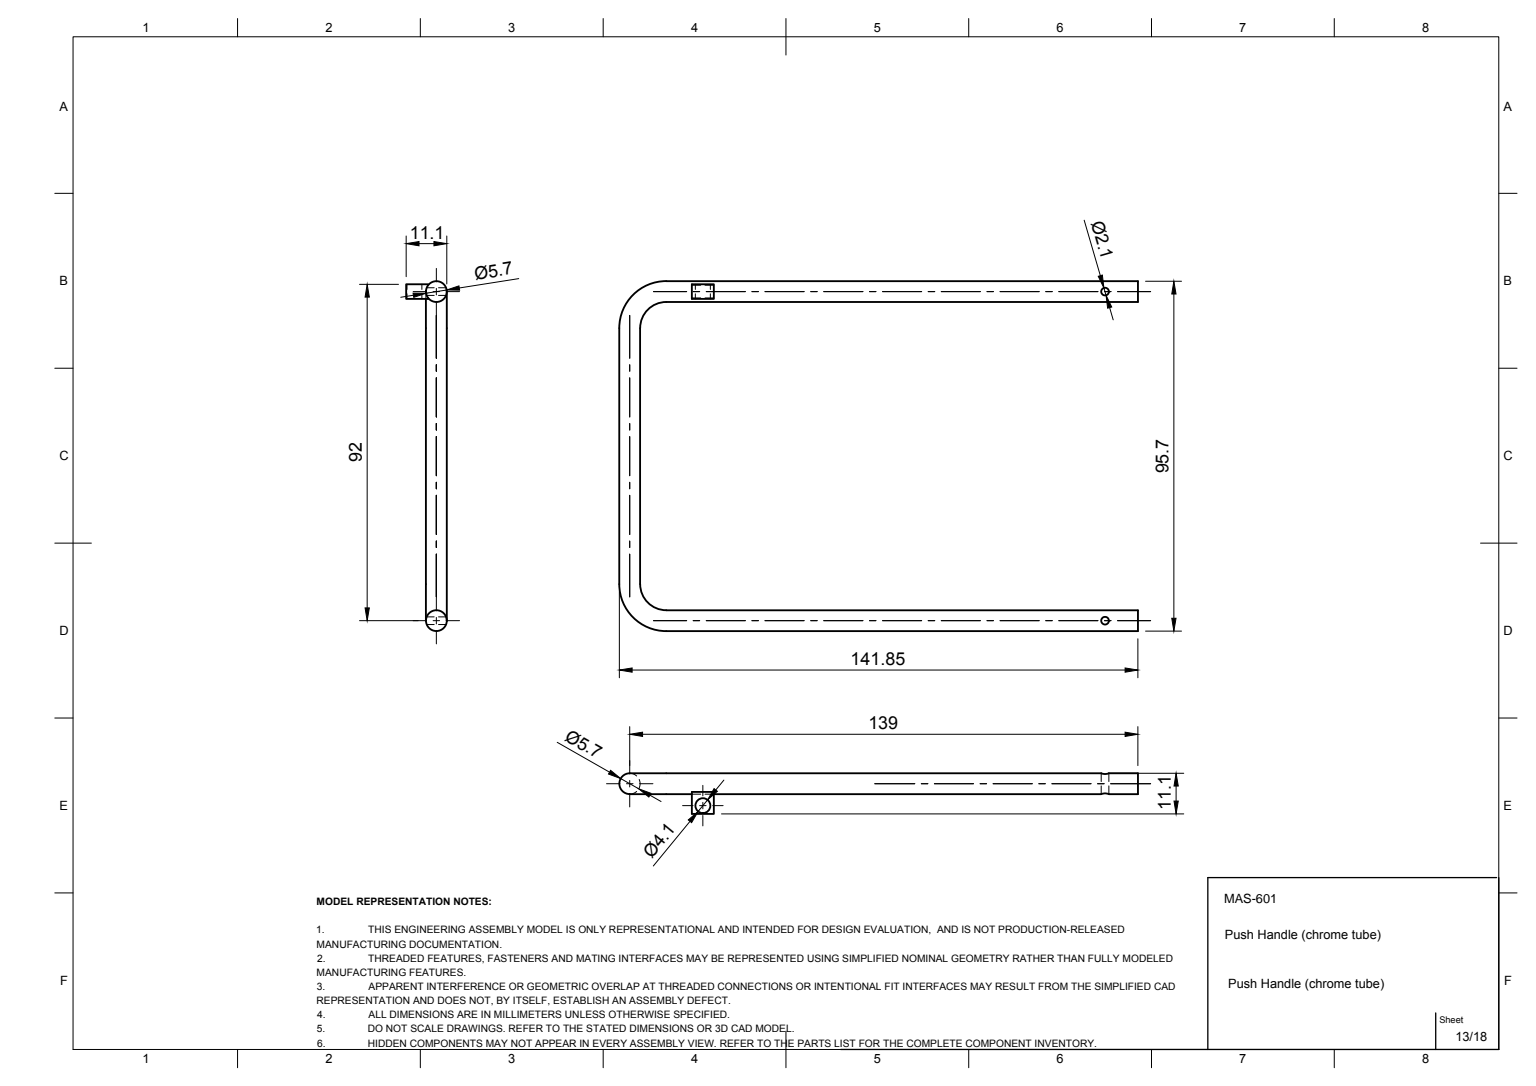
ISO-10303-21;
HEADER;
FILE_DESCRIPTION((''),'2;1');
FILE_NAME('Push Handle (chrome tube).step','2026-10-06T07:37:42+05:00',(''),(''),'','','');
FILE_SCHEMA (('AUTOMOTIVE_DESIGN { 1 0 10303 214 3 1 1 }'));
ENDSEC;
DATA;
#10=MECHANICAL_DESIGN_GEOMETRIC_PRESENTATION_REPRESENTATION('',(#381),#18757);
#335=TOROIDAL_SURFACE('',#10190,10.,2.85) ;
#336=TOROIDAL_SURFACE('',#10197,10.,2.85) ;
#347=SHAPE_REPRESENTATION_RELATIONSHIP('SRR','None',#18865,#364) ;
#364=ADVANCED_BREP_SHAPE_REPRESENTATION('',(#398),#18748) ;
#381=STYLED_ITEM('',(#18959),#398) ;
#398=MANIFOLD_SOLID_BREP('Push Handle (chrome tube)',#9550) ;
#428=B_SPLINE_CURVE_WITH_KNOTS('',3,(#14926,#14927,#14928,#14929,#14930,
#14931,#14932,#14933,#14934,#14935,#14936,#14937,#14938,#14939,#14940,#14941,
#14942,#14943),.UNSPECIFIED.,.F.,.F.,(4,2,2,2,2,2,2,2,4),(0.159853073606258,
0.199802153604227,0.239751233602197,0.279728690407356,0.319706147212516,
0.359683604017676,0.399661060822836,0.439610140820805,0.479559220818774),
 .UNSPECIFIED.) ;
#429=B_SPLINE_CURVE_WITH_KNOTS('',3,(#14944,#14945,#14946,#14947,#14948,
#14949,#14950,#14951,#14952,#14953,#14954,#14955,#14956,#14957,#14958,#14959,
#14960,#14961,#14962),.UNSPECIFIED.,.F.,.F.,(4,2,2,2,3,2,2,2,4),(0.479559220818774,
0.519508300816743,0.559457380814712,0.599434837619873,0.639412294425033,
0.679389751230192,0.719367208035352,0.759316288033321,0.799265368031291),
 .UNSPECIFIED.) ;
#430=B_SPLINE_CURVE_WITH_KNOTS('',3,(#14966,#14967,#14968,#14969,#14970,
#14971,#14972,#14973,#14974,#14975,#14976,#14977,#14978,#14979,#14980,#14981,
#14982,#14983,#14984),.UNSPECIFIED.,.F.,.F.,(4,2,2,2,3,2,2,2,4),(0.479559220818775,
0.519508300816745,0.559457380814714,0.599434837619874,0.639412294425033,
0.679389751230193,0.719367208035354,0.759316288033323,0.799265368031292),
 .UNSPECIFIED.) ;
#431=B_SPLINE_CURVE_WITH_KNOTS('',3,(#14985,#14986,#14987,#14988,#14989,
#14990,#14991,#14992,#14993,#14994,#14995,#14996,#14997,#14998,#14999,#15000,
#15001,#15002),.UNSPECIFIED.,.F.,.F.,(4,2,2,2,2,2,2,2,4),(0.159853073606259,
0.199802153604228,0.239751233602197,0.279728690407357,0.319706147212517,
0.359683604017677,0.399661060822836,0.439610140820806,0.479559220818775),
 .UNSPECIFIED.) ;
#432=B_SPLINE_CURVE_WITH_KNOTS('',3,(#15006,#15007,#15008,#15009,#15010,
#15011,#15012,#15013,#15014,#15015,#15016,#15017,#15018,#15019,#15020,#15021,
#15022,#15023),.UNSPECIFIED.,.F.,.F.,(4,2,2,2,2,2,2,2,4),(0.159853073606258,
0.199802153604227,0.239751233602197,0.279728690407356,0.319706147212516,
0.359683604017676,0.399661060822836,0.439610140820805,0.479559220818774),
 .UNSPECIFIED.) ;
#433=B_SPLINE_CURVE_WITH_KNOTS('',3,(#15027,#15028,#15029,#15030,#15031,
#15032,#15033,#15034,#15035,#15036,#15037,#15038,#15039,#15040,#15041,#15042,
#15043,#15044),.UNSPECIFIED.,.F.,.F.,(4,2,2,2,2,2,2,2,4),(0.159853073606258,
0.199802153604227,0.239751233602197,0.279728690407356,0.319706147212516,
0.359683604017676,0.399661060822836,0.439610140820805,0.479559220818774),
 .UNSPECIFIED.) ;
#434=B_SPLINE_CURVE_WITH_KNOTS('',3,(#15045,#15046,#15047,#15048,#15049,
#15050,#15051,#15052,#15053,#15054,#15055,#15056,#15057,#15058,#15059,#15060,
#15061,#15062,#15063),.UNSPECIFIED.,.F.,.F.,(4,2,2,2,3,2,2,2,4),(0.479559220818774,
0.519508300816744,0.559457380814713,0.599434837619873,0.639412294425033,
0.679389751230192,0.719367208035352,0.759316288033321,0.799265368031291),
 .UNSPECIFIED.) ;
#435=B_SPLINE_CURVE_WITH_KNOTS('',3,(#15064,#15065,#15066,#15067,#15068,
#15069,#15070,#15071,#15072,#15073,#15074,#15075,#15076,#15077,#15078,#15079,
#15080,#15081,#15082),.UNSPECIFIED.,.F.,.F.,(4,2,2,2,3,2,2,2,4),(0.479559220818774,
0.519508300816744,0.559457380814713,0.599434837619873,0.639412294425033,
0.679389751230192,0.719367208035352,0.759316288033321,0.799265368031291),
 .UNSPECIFIED.) ;
#579=CYLINDRICAL_SURFACE('',#10172,1.05) ;
#580=CYLINDRICAL_SURFACE('',#10173,1.05) ;
#581=CYLINDRICAL_SURFACE('',#10174,2.05) ;
#582=CYLINDRICAL_SURFACE('',#10186,2.85) ;
#583=CYLINDRICAL_SURFACE('',#10194,2.85) ;
#584=CYLINDRICAL_SURFACE('',#10201,2.85) ;
#722=FACE_BOUND('',#1917,.T.) ;
#723=FACE_BOUND('',#1920,.T.) ;
#724=FACE_BOUND('',#1924,.T.) ;
#725=FACE_BOUND('',#1929,.T.) ;
#726=FACE_BOUND('',#1930,.T.) ;
#893=PLANE('',#10177) ;
#894=PLANE('',#10179) ;
#895=PLANE('',#10180) ;
#896=PLANE('',#10181) ;
#897=PLANE('',#10182) ;
#898=PLANE('',#10183) ;
#899=PLANE('',#10184) ;
#900=PLANE('',#10203) ;
#901=PLANE('',#10204) ;
#1321=FACE_OUTER_BOUND('',#1911,.T.) ;
#1322=FACE_OUTER_BOUND('',#1912,.T.) ;
#1323=FACE_OUTER_BOUND('',#1913,.T.) ;
#1324=FACE_OUTER_BOUND('',#1914,.T.) ;
#1325=FACE_OUTER_BOUND('',#1915,.T.) ;
#1326=FACE_OUTER_BOUND('',#1916,.T.) ;
#1327=FACE_OUTER_BOUND('',#1918,.T.) ;
#1328=FACE_OUTER_BOUND('',#1919,.T.) ;
#1329=FACE_OUTER_BOUND('',#1921,.T.) ;
#1330=FACE_OUTER_BOUND('',#1922,.T.) ;
#1331=FACE_OUTER_BOUND('',#1923,.T.) ;
#1332=FACE_OUTER_BOUND('',#1925,.T.) ;
#1333=FACE_OUTER_BOUND('',#1926,.T.) ;
#1334=FACE_OUTER_BOUND('',#1927,.T.) ;
#1335=FACE_OUTER_BOUND('',#1928,.T.) ;
#1336=FACE_OUTER_BOUND('',#1931,.T.) ;
#1337=FACE_OUTER_BOUND('',#1932,.T.) ;
#1911=EDGE_LOOP('',(#7511,#7512,#7513,#7514,#7515,#7516)) ;
#1912=EDGE_LOOP('',(#7517,#7518,#7519,#7520,#7521,#7522)) ;
#1913=EDGE_LOOP('',(#7523,#7524,#7525,#7526)) ;
#1914=EDGE_LOOP('',(#7527,#7528,#7529,#7530,#7531,#7532)) ;
#1915=EDGE_LOOP('',(#7533,#7534,#7535,#7536)) ;
#1916=EDGE_LOOP('',(#7537,#7538,#7539,#7540)) ;
#1917=EDGE_LOOP('',(#7541)) ;
#1918=EDGE_LOOP('',(#7542,#7543,#7544,#7545)) ;
#1919=EDGE_LOOP('',(#7546,#7547,#7548,#7549)) ;
#1920=EDGE_LOOP('',(#7550)) ;
#1921=EDGE_LOOP('',(#7551,#7552,#7553,#7554)) ;
#1922=EDGE_LOOP('',(#7555,#7556,#7557,#7558,#7559,#7560)) ;
#1923=EDGE_LOOP('',(#7561,#7562,#7563,#7564,#7565,#7566,#7567,#7568,#7569)) ;
#1924=EDGE_LOOP('',(#7570,#7571)) ;
#1925=EDGE_LOOP('',(#7572,#7573,#7574,#7575,#7576,#7577)) ;
#1926=EDGE_LOOP('',(#7578,#7579,#7580,#7581,#7582,#7583)) ;
#1927=EDGE_LOOP('',(#7584,#7585,#7586,#7587,#7588,#7589)) ;
#1928=EDGE_LOOP('',(#7590,#7591,#7592,#7593,#7594,#7595,#7596,#7597,#7598)) ;
#1929=EDGE_LOOP('',(#7599,#7600)) ;
#1930=EDGE_LOOP('',(#7601,#7602,#7603,#7604)) ;
#1931=EDGE_LOOP('',(#7605)) ;
#1932=EDGE_LOOP('',(#7606)) ;
#2613=LINE('',#14964,#3384) ;
#2614=LINE('',#15025,#3385) ;
#2615=LINE('',#15087,#3386) ;
#2616=LINE('',#15094,#3387) ;
#2617=LINE('',#15096,#3388) ;
#2618=LINE('',#15098,#3389) ;
#2619=LINE('',#15100,#3390) ;
#2620=LINE('',#15101,#3391) ;
#2621=LINE('',#15104,#3392) ;
#2622=LINE('',#15106,#3393) ;
#2623=LINE('',#15107,#3394) ;
#2624=LINE('',#15111,#3395) ;
#2625=LINE('',#15112,#3396) ;
#2626=LINE('',#15113,#3397) ;
#2627=LINE('',#15116,#3398) ;
#2628=LINE('',#15117,#3399) ;
#2629=LINE('',#15119,#3400) ;
#2630=LINE('',#15122,#3401) ;
#2631=LINE('',#15123,#3402) ;
#2632=LINE('',#15129,#3403) ;
#2633=LINE('',#15131,#3404) ;
#2634=LINE('',#15143,#3405) ;
#2635=LINE('',#15154,#3406) ;
#2636=LINE('',#15156,#3407) ;
#3384=VECTOR('',#11947,1.05) ;
#3385=VECTOR('',#11950,1.05) ;
#3386=VECTOR('',#11955,2.05) ;
#3387=VECTOR('',#11962,10.) ;
#3388=VECTOR('',#11963,10.) ;
#3389=VECTOR('',#11964,10.) ;
#3390=VECTOR('',#11965,10.) ;
#3391=VECTOR('',#11966,10.) ;
#3392=VECTOR('',#11969,10.) ;
#3393=VECTOR('',#11970,10.) ;
#3394=VECTOR('',#11971,10.) ;
#3395=VECTOR('',#11974,10.) ;
#3396=VECTOR('',#11975,10.) ;
#3397=VECTOR('',#11976,10.) ;
#3398=VECTOR('',#11979,10.) ;
#3399=VECTOR('',#11980,10.) ;
#3400=VECTOR('',#11983,10.) ;
#3401=VECTOR('',#11986,10.) ;
#3402=VECTOR('',#11987,10.) ;
#3403=VECTOR('',#11996,2.85) ;
#3404=VECTOR('',#11997,2.85) ;
#3405=VECTOR('',#12012,2.85) ;
#3406=VECTOR('',#12027,2.85) ;
#3407=VECTOR('',#12028,2.85) ;
#3956=CIRCLE('',#10175,2.05) ;
#3957=CIRCLE('',#10176,2.05) ;
#3958=CIRCLE('',#10178,2.85) ;
#3959=CIRCLE('',#10185,2.85) ;
#3960=CIRCLE('',#10187,2.85) ;
#3961=CIRCLE('',#10188,2.85) ;
#3962=CIRCLE('',#10189,2.85) ;
#3963=CIRCLE('',#10191,7.15) ;
#3964=CIRCLE('',#10192,2.85) ;
#3965=CIRCLE('',#10193,2.85) ;
#3966=CIRCLE('',#10195,2.85) ;
#3967=CIRCLE('',#10196,2.85) ;
#3968=CIRCLE('',#10198,7.15000000000003) ;
#3969=CIRCLE('',#10199,2.85) ;
#3970=CIRCLE('',#10200,2.85) ;
#3971=CIRCLE('',#10202,2.85) ;
#4533=VERTEX_POINT('',#14924) ;
#4534=VERTEX_POINT('',#14925) ;
#4535=VERTEX_POINT('',#14963) ;
#4536=VERTEX_POINT('',#14965) ;
#4537=VERTEX_POINT('',#15004) ;
#4538=VERTEX_POINT('',#15005) ;
#4539=VERTEX_POINT('',#15024) ;
#4540=VERTEX_POINT('',#15026) ;
#4541=VERTEX_POINT('',#15084) ;
#4542=VERTEX_POINT('',#15086) ;
#4543=VERTEX_POINT('',#15090) ;
#4544=VERTEX_POINT('',#15091) ;
#4545=VERTEX_POINT('',#15093) ;
#4546=VERTEX_POINT('',#15095) ;
#4547=VERTEX_POINT('',#15097) ;
#4548=VERTEX_POINT('',#15099) ;
#4549=VERTEX_POINT('',#15103) ;
#4550=VERTEX_POINT('',#15105) ;
#4551=VERTEX_POINT('',#15109) ;
#4552=VERTEX_POINT('',#15110) ;
#4553=VERTEX_POINT('',#15115) ;
#4554=VERTEX_POINT('',#15121) ;
#4555=VERTEX_POINT('',#15127) ;
#4556=VERTEX_POINT('',#15130) ;
#4557=VERTEX_POINT('',#15132) ;
#4558=VERTEX_POINT('',#15136) ;
#4559=VERTEX_POINT('',#15138) ;
#4560=VERTEX_POINT('',#15142) ;
#4561=VERTEX_POINT('',#15144) ;
#4562=VERTEX_POINT('',#15148) ;
#4563=VERTEX_POINT('',#15150) ;
#4564=VERTEX_POINT('',#15155) ;
#5602=EDGE_CURVE('',#4533,#4534,#428,.T.) ;
#5603=EDGE_CURVE('',#4534,#4533,#429,.T.) ;
#5604=EDGE_CURVE('',#4534,#4535,#2613,.T.) ;
#5605=EDGE_CURVE('',#4536,#4535,#430,.T.) ;
#5606=EDGE_CURVE('',#4535,#4536,#431,.T.) ;
#5607=EDGE_CURVE('',#4537,#4538,#432,.T.) ;
#5608=EDGE_CURVE('',#4537,#4539,#2614,.T.) ;
#5609=EDGE_CURVE('',#4540,#4539,#433,.T.) ;
#5610=EDGE_CURVE('',#4539,#4540,#434,.T.) ;
#5611=EDGE_CURVE('',#4538,#4537,#435,.T.) ;
#5612=EDGE_CURVE('',#4541,#4541,#3956,.T.) ;
#5613=EDGE_CURVE('',#4541,#4542,#2615,.T.) ;
#5614=EDGE_CURVE('',#4542,#4542,#3957,.T.) ;
#5615=EDGE_CURVE('',#4543,#4544,#3958,.T.) ;
#5616=EDGE_CURVE('',#4543,#4545,#2616,.T.) ;
#5617=EDGE_CURVE('',#4545,#4546,#2617,.T.) ;
#5618=EDGE_CURVE('',#4546,#4547,#2618,.T.) ;
#5619=EDGE_CURVE('',#4547,#4548,#2619,.T.) ;
#5620=EDGE_CURVE('',#4548,#4544,#2620,.T.) ;
#5621=EDGE_CURVE('',#4549,#4543,#2621,.T.) ;
#5622=EDGE_CURVE('',#4549,#4550,#2622,.T.) ;
#5623=EDGE_CURVE('',#4550,#4545,#2623,.T.) ;
#5624=EDGE_CURVE('',#4551,#4552,#2624,.T.) ;
#5625=EDGE_CURVE('',#4552,#4548,#2625,.T.) ;
#5626=EDGE_CURVE('',#4551,#4547,#2626,.T.) ;
#5627=EDGE_CURVE('',#4553,#4551,#2627,.T.) ;
#5628=EDGE_CURVE('',#4553,#4546,#2628,.T.) ;
#5629=EDGE_CURVE('',#4550,#4553,#2629,.T.) ;
#5630=EDGE_CURVE('',#4544,#4554,#2630,.T.) ;
#5631=EDGE_CURVE('',#4552,#4554,#2631,.T.) ;
#5632=EDGE_CURVE('',#4554,#4549,#3959,.T.) ;
#5633=EDGE_CURVE('',#4555,#4555,#3960,.T.) ;
#5634=EDGE_CURVE('',#4555,#4536,#2632,.T.) ;
#5635=EDGE_CURVE('',#4535,#4556,#2633,.T.) ;
#5636=EDGE_CURVE('',#4556,#4557,#3961,.T.) ;
#5637=EDGE_CURVE('',#4557,#4556,#3962,.T.) ;
#5638=EDGE_CURVE('',#4557,#4558,#3963,.T.) ;
#5639=EDGE_CURVE('',#4558,#4559,#3964,.T.) ;
#5640=EDGE_CURVE('',#4559,#4558,#3965,.T.) ;
#5641=EDGE_CURVE('',#4559,#4560,#2634,.T.) ;
#5642=EDGE_CURVE('',#4560,#4561,#3966,.T.) ;
#5643=EDGE_CURVE('',#4561,#4560,#3967,.T.) ;
#5644=EDGE_CURVE('',#4561,#4562,#3968,.T.) ;
#5645=EDGE_CURVE('',#4562,#4563,#3969,.T.) ;
#5646=EDGE_CURVE('',#4563,#4562,#3970,.T.) ;
#5647=EDGE_CURVE('',#4563,#4539,#2635,.T.) ;
#5648=EDGE_CURVE('',#4540,#4564,#2636,.T.) ;
#5649=EDGE_CURVE('',#4564,#4564,#3971,.T.) ;
#7511=ORIENTED_EDGE('',*,*,#5602,.F.) ;
#7512=ORIENTED_EDGE('',*,*,#5603,.F.) ;
#7513=ORIENTED_EDGE('',*,*,#5604,.T.) ;
#7514=ORIENTED_EDGE('',*,*,#5605,.F.) ;
#7515=ORIENTED_EDGE('',*,*,#5606,.F.) ;
#7516=ORIENTED_EDGE('',*,*,#5604,.F.) ;
#7517=ORIENTED_EDGE('',*,*,#5607,.F.) ;
#7518=ORIENTED_EDGE('',*,*,#5608,.T.) ;
#7519=ORIENTED_EDGE('',*,*,#5609,.F.) ;
#7520=ORIENTED_EDGE('',*,*,#5610,.F.) ;
#7521=ORIENTED_EDGE('',*,*,#5608,.F.) ;
#7522=ORIENTED_EDGE('',*,*,#5611,.F.) ;
#7523=ORIENTED_EDGE('',*,*,#5612,.F.) ;
#7524=ORIENTED_EDGE('',*,*,#5613,.T.) ;
#7525=ORIENTED_EDGE('',*,*,#5614,.F.) ;
#7526=ORIENTED_EDGE('',*,*,#5613,.F.) ;
#7527=ORIENTED_EDGE('',*,*,#5615,.F.) ;
#7528=ORIENTED_EDGE('',*,*,#5616,.T.) ;
#7529=ORIENTED_EDGE('',*,*,#5617,.T.) ;
#7530=ORIENTED_EDGE('',*,*,#5618,.T.) ;
#7531=ORIENTED_EDGE('',*,*,#5619,.T.) ;
#7532=ORIENTED_EDGE('',*,*,#5620,.T.) ;
#7533=ORIENTED_EDGE('',*,*,#5621,.F.) ;
#7534=ORIENTED_EDGE('',*,*,#5622,.T.) ;
#7535=ORIENTED_EDGE('',*,*,#5623,.T.) ;
#7536=ORIENTED_EDGE('',*,*,#5616,.F.) ;
#7537=ORIENTED_EDGE('',*,*,#5624,.T.) ;
#7538=ORIENTED_EDGE('',*,*,#5625,.T.) ;
#7539=ORIENTED_EDGE('',*,*,#5619,.F.) ;
#7540=ORIENTED_EDGE('',*,*,#5626,.F.) ;
#7541=ORIENTED_EDGE('',*,*,#5614,.T.) ;
#7542=ORIENTED_EDGE('',*,*,#5627,.T.) ;
#7543=ORIENTED_EDGE('',*,*,#5626,.T.) ;
#7544=ORIENTED_EDGE('',*,*,#5618,.F.) ;
#7545=ORIENTED_EDGE('',*,*,#5628,.F.) ;
#7546=ORIENTED_EDGE('',*,*,#5629,.T.) ;
#7547=ORIENTED_EDGE('',*,*,#5628,.T.) ;
#7548=ORIENTED_EDGE('',*,*,#5617,.F.) ;
#7549=ORIENTED_EDGE('',*,*,#5623,.F.) ;
#7550=ORIENTED_EDGE('',*,*,#5612,.T.) ;
#7551=ORIENTED_EDGE('',*,*,#5630,.F.) ;
#7552=ORIENTED_EDGE('',*,*,#5620,.F.) ;
#7553=ORIENTED_EDGE('',*,*,#5625,.F.) ;
#7554=ORIENTED_EDGE('',*,*,#5631,.T.) ;
#7555=ORIENTED_EDGE('',*,*,#5632,.F.) ;
#7556=ORIENTED_EDGE('',*,*,#5631,.F.) ;
#7557=ORIENTED_EDGE('',*,*,#5624,.F.) ;
#7558=ORIENTED_EDGE('',*,*,#5627,.F.) ;
#7559=ORIENTED_EDGE('',*,*,#5629,.F.) ;
#7560=ORIENTED_EDGE('',*,*,#5622,.F.) ;
#7561=ORIENTED_EDGE('',*,*,#5633,.F.) ;
#7562=ORIENTED_EDGE('',*,*,#5634,.T.) ;
#7563=ORIENTED_EDGE('',*,*,#5605,.T.) ;
#7564=ORIENTED_EDGE('',*,*,#5635,.T.) ;
#7565=ORIENTED_EDGE('',*,*,#5636,.T.) ;
#7566=ORIENTED_EDGE('',*,*,#5637,.T.) ;
#7567=ORIENTED_EDGE('',*,*,#5635,.F.) ;
#7568=ORIENTED_EDGE('',*,*,#5606,.T.) ;
#7569=ORIENTED_EDGE('',*,*,#5634,.F.) ;
#7570=ORIENTED_EDGE('',*,*,#5602,.T.) ;
#7571=ORIENTED_EDGE('',*,*,#5603,.T.) ;
#7572=ORIENTED_EDGE('',*,*,#5636,.F.) ;
#7573=ORIENTED_EDGE('',*,*,#5637,.F.) ;
#7574=ORIENTED_EDGE('',*,*,#5638,.T.) ;
#7575=ORIENTED_EDGE('',*,*,#5639,.T.) ;
#7576=ORIENTED_EDGE('',*,*,#5640,.T.) ;
#7577=ORIENTED_EDGE('',*,*,#5638,.F.) ;
#7578=ORIENTED_EDGE('',*,*,#5640,.F.) ;
#7579=ORIENTED_EDGE('',*,*,#5641,.T.) ;
#7580=ORIENTED_EDGE('',*,*,#5642,.T.) ;
#7581=ORIENTED_EDGE('',*,*,#5643,.T.) ;
#7582=ORIENTED_EDGE('',*,*,#5641,.F.) ;
#7583=ORIENTED_EDGE('',*,*,#5639,.F.) ;
#7584=ORIENTED_EDGE('',*,*,#5642,.F.) ;
#7585=ORIENTED_EDGE('',*,*,#5643,.F.) ;
#7586=ORIENTED_EDGE('',*,*,#5644,.T.) ;
#7587=ORIENTED_EDGE('',*,*,#5645,.T.) ;
#7588=ORIENTED_EDGE('',*,*,#5646,.T.) ;
#7589=ORIENTED_EDGE('',*,*,#5644,.F.) ;
#7590=ORIENTED_EDGE('',*,*,#5646,.F.) ;
#7591=ORIENTED_EDGE('',*,*,#5647,.T.) ;
#7592=ORIENTED_EDGE('',*,*,#5610,.T.) ;
#7593=ORIENTED_EDGE('',*,*,#5648,.T.) ;
#7594=ORIENTED_EDGE('',*,*,#5649,.T.) ;
#7595=ORIENTED_EDGE('',*,*,#5648,.F.) ;
#7596=ORIENTED_EDGE('',*,*,#5609,.T.) ;
#7597=ORIENTED_EDGE('',*,*,#5647,.F.) ;
#7598=ORIENTED_EDGE('',*,*,#5645,.F.) ;
#7599=ORIENTED_EDGE('',*,*,#5607,.T.) ;
#7600=ORIENTED_EDGE('',*,*,#5611,.T.) ;
#7601=ORIENTED_EDGE('',*,*,#5621,.T.) ;
#7602=ORIENTED_EDGE('',*,*,#5615,.T.) ;
#7603=ORIENTED_EDGE('',*,*,#5630,.T.) ;
#7604=ORIENTED_EDGE('',*,*,#5632,.T.) ;
#7605=ORIENTED_EDGE('',*,*,#5633,.T.) ;
#7606=ORIENTED_EDGE('',*,*,#5649,.F.) ;
#9257=ADVANCED_FACE('',(#1321),#579,.F.) ;
#9258=ADVANCED_FACE('',(#1322),#580,.F.) ;
#9259=ADVANCED_FACE('',(#1323),#581,.F.) ;
#9260=ADVANCED_FACE('',(#1324),#893,.T.) ;
#9261=ADVANCED_FACE('',(#1325),#894,.T.) ;
#9262=ADVANCED_FACE('',(#1326,#722),#895,.T.) ;
#9263=ADVANCED_FACE('',(#1327),#896,.T.) ;
#9264=ADVANCED_FACE('',(#1328,#723),#897,.T.) ;
#9265=ADVANCED_FACE('',(#1329),#898,.T.) ;
#9266=ADVANCED_FACE('',(#1330),#899,.F.) ;
#9267=ADVANCED_FACE('',(#1331,#724),#582,.T.) ;
#9268=ADVANCED_FACE('',(#1332),#335,.T.) ;
#9269=ADVANCED_FACE('',(#1333),#583,.T.) ;
#9270=ADVANCED_FACE('',(#1334),#336,.T.) ;
#9271=ADVANCED_FACE('',(#1335,#725,#726),#584,.T.) ;
#9272=ADVANCED_FACE('',(#1336),#900,.T.) ;
#9273=ADVANCED_FACE('',(#1337),#901,.F.) ;
#9550=CLOSED_SHELL('',(#9257,#9258,#9259,#9260,#9261,#9262,#9263,#9264,
#9265,#9266,#9267,#9268,#9269,#9270,#9271,#9272,#9273)) ;
#10171=AXIS2_PLACEMENT_3D('',#14922,#11943,#11944) ;
#10172=AXIS2_PLACEMENT_3D('',#14923,#11945,#11946) ;
#10173=AXIS2_PLACEMENT_3D('',#15003,#11948,#11949) ;
#10174=AXIS2_PLACEMENT_3D('',#15083,#11951,#11952) ;
#10175=AXIS2_PLACEMENT_3D('',#15085,#11953,#11954) ;
#10176=AXIS2_PLACEMENT_3D('',#15088,#11956,#11957) ;
#10177=AXIS2_PLACEMENT_3D('',#15089,#11958,#11959) ;
#10178=AXIS2_PLACEMENT_3D('',#15092,#11960,#11961) ;
#10179=AXIS2_PLACEMENT_3D('',#15102,#11967,#11968) ;
#10180=AXIS2_PLACEMENT_3D('',#15108,#11972,#11973) ;
#10181=AXIS2_PLACEMENT_3D('',#15114,#11977,#11978) ;
#10182=AXIS2_PLACEMENT_3D('',#15118,#11981,#11982) ;
#10183=AXIS2_PLACEMENT_3D('',#15120,#11984,#11985) ;
#10184=AXIS2_PLACEMENT_3D('',#15124,#11988,#11989) ;
#10185=AXIS2_PLACEMENT_3D('',#15125,#11990,#11991) ;
#10186=AXIS2_PLACEMENT_3D('',#15126,#11992,#11993) ;
#10187=AXIS2_PLACEMENT_3D('',#15128,#11994,#11995) ;
#10188=AXIS2_PLACEMENT_3D('',#15133,#11998,#11999) ;
#10189=AXIS2_PLACEMENT_3D('',#15134,#12000,#12001) ;
#10190=AXIS2_PLACEMENT_3D('',#15135,#12002,#12003) ;
#10191=AXIS2_PLACEMENT_3D('',#15137,#12004,#12005) ;
#10192=AXIS2_PLACEMENT_3D('',#15139,#12006,#12007) ;
#10193=AXIS2_PLACEMENT_3D('',#15140,#12008,#12009) ;
#10194=AXIS2_PLACEMENT_3D('',#15141,#12010,#12011) ;
#10195=AXIS2_PLACEMENT_3D('',#15145,#12013,#12014) ;
#10196=AXIS2_PLACEMENT_3D('',#15146,#12015,#12016) ;
#10197=AXIS2_PLACEMENT_3D('',#15147,#12017,#12018) ;
#10198=AXIS2_PLACEMENT_3D('',#15149,#12019,#12020) ;
#10199=AXIS2_PLACEMENT_3D('',#15151,#12021,#12022) ;
#10200=AXIS2_PLACEMENT_3D('',#15152,#12023,#12024) ;
#10201=AXIS2_PLACEMENT_3D('',#15153,#12025,#12026) ;
#10202=AXIS2_PLACEMENT_3D('',#15157,#12029,#12030) ;
#10203=AXIS2_PLACEMENT_3D('',#15158,#12031,#12032) ;
#10204=AXIS2_PLACEMENT_3D('',#15159,#12033,#12034) ;
#11943=DIRECTION('axis',(0.,0.,1.)) ;
#11944=DIRECTION('refdir',(1.,0.,0.)) ;
#11945=DIRECTION('center_axis',(-1.,0.,0.)) ;
#11946=DIRECTION('ref_axis',(0.,0.,-1.)) ;
#11947=DIRECTION('',(-1.,0.,0.)) ;
#11948=DIRECTION('center_axis',(-1.,0.,0.)) ;
#11949=DIRECTION('ref_axis',(0.,0.,-1.)) ;
#11950=DIRECTION('',(-1.,0.,0.)) ;
#11951=DIRECTION('center_axis',(0.,1.,0.)) ;
#11952=DIRECTION('ref_axis',(1.,0.,0.)) ;
#11953=DIRECTION('center_axis',(0.,1.,0.)) ;
#11954=DIRECTION('ref_axis',(1.,0.,0.)) ;
#11955=DIRECTION('',(0.,1.,0.)) ;
#11956=DIRECTION('center_axis',(0.,-1.,0.)) ;
#11957=DIRECTION('ref_axis',(1.,0.,0.)) ;
#11958=DIRECTION('center_axis',(0.,0.,1.)) ;
#11959=DIRECTION('ref_axis',(1.,0.,0.)) ;
#11960=DIRECTION('center_axis',(0.,0.,1.)) ;
#11961=DIRECTION('ref_axis',(1.,0.,0.)) ;
#11962=DIRECTION('',(0.,-1.,0.)) ;
#11963=DIRECTION('',(1.,0.,0.)) ;
#11964=DIRECTION('',(0.,1.,0.)) ;
#11965=DIRECTION('',(-1.,0.,0.)) ;
#11966=DIRECTION('',(0.,-1.,0.)) ;
#11967=DIRECTION('center_axis',(-1.,0.,0.)) ;
#11968=DIRECTION('ref_axis',(0.,-1.,0.)) ;
#11969=DIRECTION('',(0.,0.,1.)) ;
#11970=DIRECTION('',(0.,-1.,0.)) ;
#11971=DIRECTION('',(0.,0.,1.)) ;
#11972=DIRECTION('center_axis',(0.,1.,0.)) ;
#11973=DIRECTION('ref_axis',(-1.,0.,0.)) ;
#11974=DIRECTION('',(-1.,0.,0.)) ;
#11975=DIRECTION('',(0.,0.,1.)) ;
#11976=DIRECTION('',(0.,0.,1.)) ;
#11977=DIRECTION('center_axis',(1.,0.,0.)) ;
#11978=DIRECTION('ref_axis',(0.,1.,0.)) ;
#11979=DIRECTION('',(0.,1.,0.)) ;
#11980=DIRECTION('',(0.,0.,1.)) ;
#11981=DIRECTION('center_axis',(0.,-1.,0.)) ;
#11982=DIRECTION('ref_axis',(1.,0.,0.)) ;
#11983=DIRECTION('',(1.,0.,0.)) ;
#11984=DIRECTION('center_axis',(-1.,0.,0.)) ;
#11985=DIRECTION('ref_axis',(0.,-1.,0.)) ;
#11986=DIRECTION('',(0.,0.,-1.)) ;
#11987=DIRECTION('',(0.,-1.,0.)) ;
#11988=DIRECTION('center_axis',(0.,0.,1.)) ;
#11989=DIRECTION('ref_axis',(1.,0.,0.)) ;
#11990=DIRECTION('center_axis',(0.,0.,-1.)) ;
#11991=DIRECTION('ref_axis',(1.,0.,0.)) ;
#11992=DIRECTION('center_axis',(0.,0.,-1.)) ;
#11993=DIRECTION('ref_axis',(1.,0.,0.)) ;
#11994=DIRECTION('center_axis',(0.,-3.67517835871524E-15,-1.)) ;
#11995=DIRECTION('ref_axis',(1.,0.,0.)) ;
#11996=DIRECTION('',(0.,0.,1.)) ;
#11997=DIRECTION('',(0.,0.,1.)) ;
#11998=DIRECTION('center_axis',(0.,-3.67517835871524E-15,-1.)) ;
#11999=DIRECTION('ref_axis',(1.,0.,0.)) ;
#12000=DIRECTION('center_axis',(0.,-3.67517835871524E-15,-1.)) ;
#12001=DIRECTION('ref_axis',(1.,0.,0.)) ;
#12002=DIRECTION('center_axis',(1.,0.,0.)) ;
#12003=DIRECTION('ref_axis',(0.,0.,-1.)) ;
#12004=DIRECTION('center_axis',(-1.,0.,0.)) ;
#12005=DIRECTION('ref_axis',(0.,0.,-1.)) ;
#12006=DIRECTION('center_axis',(0.,-1.,1.83758917935762E-15)) ;
#12007=DIRECTION('ref_axis',(1.,0.,0.)) ;
#12008=DIRECTION('center_axis',(0.,-1.,1.83758917935762E-15)) ;
#12009=DIRECTION('ref_axis',(1.,0.,0.)) ;
#12010=DIRECTION('center_axis',(0.,-1.,0.)) ;
#12011=DIRECTION('ref_axis',(1.,0.,0.)) ;
#12012=DIRECTION('',(0.,1.,0.)) ;
#12013=DIRECTION('center_axis',(0.,-1.,1.83758917935762E-15)) ;
#12014=DIRECTION('ref_axis',(1.,0.,0.)) ;
#12015=DIRECTION('center_axis',(0.,-1.,1.83758917935762E-15)) ;
#12016=DIRECTION('ref_axis',(1.,0.,0.)) ;
#12017=DIRECTION('center_axis',(1.,0.,0.)) ;
#12018=DIRECTION('ref_axis',(0.,0.,-1.)) ;
#12019=DIRECTION('center_axis',(-1.,0.,0.)) ;
#12020=DIRECTION('ref_axis',(0.,0.,-1.)) ;
#12021=DIRECTION('center_axis',(0.,0.,1.)) ;
#12022=DIRECTION('ref_axis',(1.,0.,0.)) ;
#12023=DIRECTION('center_axis',(0.,0.,1.)) ;
#12024=DIRECTION('ref_axis',(1.,0.,0.)) ;
#12025=DIRECTION('center_axis',(0.,0.,1.)) ;
#12026=DIRECTION('ref_axis',(1.,0.,0.)) ;
#12027=DIRECTION('',(0.,0.,-1.)) ;
#12028=DIRECTION('',(0.,0.,-1.)) ;
#12029=DIRECTION('center_axis',(0.,0.,1.)) ;
#12030=DIRECTION('ref_axis',(1.,0.,0.)) ;
#12031=DIRECTION('center_axis',(0.,-3.67517835871524E-15,-1.)) ;
#12032=DIRECTION('ref_axis',(1.,0.,0.)) ;
#12033=DIRECTION('center_axis',(0.,0.,1.)) ;
#12034=DIRECTION('ref_axis',(1.,0.,0.)) ;
#14922=CARTESIAN_POINT('',(0.,0.,0.)) ;
#14923=CARTESIAN_POINT('Origin',(87.1,-45.,50.)) ;
#14924=CARTESIAN_POINT('',(87.1,-45.,48.95)) ;
#14925=CARTESIAN_POINT('',(87.1,-45.,51.05)) ;
#14926=CARTESIAN_POINT('Ctrl Pts',(87.1,-45.,48.95)) ;
#14927=CARTESIAN_POINT('Ctrl Pts',(87.1,-45.1331635999932,48.95)) ;
#14928=CARTESIAN_POINT('Ctrl Pts',(87.0897621937364,-45.2743704641551,48.9768675662366)) ;
#14929=CARTESIAN_POINT('Ctrl Pts',(87.0528075475038,-45.5327272469311,49.0844232537265)) ;
#14930=CARTESIAN_POINT('Ctrl Pts',(87.0265476839081,-45.6499697400254,49.1650454995336)) ;
#14931=CARTESIAN_POINT('Ctrl Pts',(86.9766154867118,-45.835020200063,49.3500959595712)) ;
#14932=CARTESIAN_POINT('Ctrl Pts',(86.9495293742091,-45.9155922350857,49.4673129257906)) ;
#14933=CARTESIAN_POINT('Ctrl Pts',(86.9106416723388,-46.0231099988203,49.725572678198)) ;
#14934=CARTESIAN_POINT('Ctrl Pts',(86.8995282598983,-46.05,49.8667418106495)) ;
#14935=CARTESIAN_POINT('Ctrl Pts',(86.8995282598983,-46.05,50.1332581893505)) ;
#14936=CARTESIAN_POINT('Ctrl Pts',(86.9106416723388,-46.0231099988203,50.274427321802)) ;
#14937=CARTESIAN_POINT('Ctrl Pts',(86.9495293742091,-45.9155922350857,50.5326870742094)) ;
#14938=CARTESIAN_POINT('Ctrl Pts',(86.9766154867118,-45.835020200063,50.6499040404288)) ;
#14939=CARTESIAN_POINT('Ctrl Pts',(87.0265476839081,-45.6499697400254,50.8349545004664)) ;
#14940=CARTESIAN_POINT('Ctrl Pts',(87.0528075475038,-45.5327272469311,50.9155767462735)) ;
#14941=CARTESIAN_POINT('Ctrl Pts',(87.0897621937364,-45.2743704641551,51.0231324337635)) ;
#14942=CARTESIAN_POINT('Ctrl Pts',(87.1,-45.1331635999932,51.05)) ;
#14943=CARTESIAN_POINT('Ctrl Pts',(87.1,-45.,51.05)) ;
#14944=CARTESIAN_POINT('Ctrl Pts',(87.1,-45.,51.05)) ;
#14945=CARTESIAN_POINT('Ctrl Pts',(87.1,-44.8668364000068,51.05)) ;
#14946=CARTESIAN_POINT('Ctrl Pts',(87.0897621937364,-44.7256295358449,51.0231324337635)) ;
#14947=CARTESIAN_POINT('Ctrl Pts',(87.0528075475038,-44.4672727530689,50.9155767462735)) ;
#14948=CARTESIAN_POINT('Ctrl Pts',(87.0265476839081,-44.3500302599746,50.8349545004664)) ;
#14949=CARTESIAN_POINT('Ctrl Pts',(86.9766154867118,-44.164979799937,50.6499040404288)) ;
#14950=CARTESIAN_POINT('Ctrl Pts',(86.9495293742091,-44.0844077649143,50.5326870742094)) ;
#14951=CARTESIAN_POINT('Ctrl Pts',(86.9106416723388,-43.9768900011798,50.274427321802)) ;
#14952=CARTESIAN_POINT('Ctrl Pts',(86.8995282598984,-43.95,50.1332581893505)) ;
#14953=CARTESIAN_POINT('Ctrl Pts',(86.8995282598984,-43.95,50.)) ;
#14954=CARTESIAN_POINT('Ctrl Pts',(86.8995282598984,-43.95,49.8667418106495)) ;
#14955=CARTESIAN_POINT('Ctrl Pts',(86.9106416723388,-43.9768900011797,49.725572678198)) ;
#14956=CARTESIAN_POINT('Ctrl Pts',(86.9495293742091,-44.0844077649143,49.4673129257906)) ;
#14957=CARTESIAN_POINT('Ctrl Pts',(86.9766154867118,-44.164979799937,49.3500959595712)) ;
#14958=CARTESIAN_POINT('Ctrl Pts',(87.0265476839081,-44.3500302599746,49.1650454995336)) ;
#14959=CARTESIAN_POINT('Ctrl Pts',(87.0528075475038,-44.4672727530689,49.0844232537265)) ;
#14960=CARTESIAN_POINT('Ctrl Pts',(87.0897621937364,-44.7256295358449,48.9768675662366)) ;
#14961=CARTESIAN_POINT('Ctrl Pts',(87.1,-44.8668364000068,48.95)) ;
#14962=CARTESIAN_POINT('Ctrl Pts',(87.1,-45.,48.95)) ;
#14963=CARTESIAN_POINT('',(81.4,-45.,51.05)) ;
#14964=CARTESIAN_POINT('',(87.1,-45.,51.05)) ;
#14965=CARTESIAN_POINT('',(81.4,-45.,48.95)) ;
#14966=CARTESIAN_POINT('Ctrl Pts',(81.4,-45.,48.95)) ;
#14967=CARTESIAN_POINT('Ctrl Pts',(81.4,-44.8668364000068,48.95)) ;
#14968=CARTESIAN_POINT('Ctrl Pts',(81.4102378062637,-44.7256295358449,48.9768675662366)) ;
#14969=CARTESIAN_POINT('Ctrl Pts',(81.4471924524962,-44.4672727530689,49.0844232537265)) ;
#14970=CARTESIAN_POINT('Ctrl Pts',(81.4734523160919,-44.3500302599746,49.1650454995336)) ;
#14971=CARTESIAN_POINT('Ctrl Pts',(81.5233845132882,-44.164979799937,49.3500959595712)) ;
#14972=CARTESIAN_POINT('Ctrl Pts',(81.5504706257909,-44.0844077649143,49.4673129257906)) ;
#14973=CARTESIAN_POINT('Ctrl Pts',(81.5893583276612,-43.9768900011797,49.725572678198)) ;
#14974=CARTESIAN_POINT('Ctrl Pts',(81.6004717401017,-43.95,49.8667418106495)) ;
#14975=CARTESIAN_POINT('Ctrl Pts',(81.6004717401017,-43.95,50.)) ;
#14976=CARTESIAN_POINT('Ctrl Pts',(81.6004717401017,-43.95,50.1332581893505)) ;
#14977=CARTESIAN_POINT('Ctrl Pts',(81.5893583276612,-43.9768900011798,50.274427321802)) ;
#14978=CARTESIAN_POINT('Ctrl Pts',(81.5504706257909,-44.0844077649143,50.5326870742094)) ;
#14979=CARTESIAN_POINT('Ctrl Pts',(81.5233845132882,-44.164979799937,50.6499040404288)) ;
#14980=CARTESIAN_POINT('Ctrl Pts',(81.4734523160919,-44.3500302599746,50.8349545004664)) ;
#14981=CARTESIAN_POINT('Ctrl Pts',(81.4471924524962,-44.4672727530689,50.9155767462735)) ;
#14982=CARTESIAN_POINT('Ctrl Pts',(81.4102378062637,-44.7256295358449,51.0231324337635)) ;
#14983=CARTESIAN_POINT('Ctrl Pts',(81.4,-44.8668364000068,51.05)) ;
#14984=CARTESIAN_POINT('Ctrl Pts',(81.4,-45.,51.05)) ;
#14985=CARTESIAN_POINT('Ctrl Pts',(81.4,-45.,51.05)) ;
#14986=CARTESIAN_POINT('Ctrl Pts',(81.4,-45.1331635999932,51.05)) ;
#14987=CARTESIAN_POINT('Ctrl Pts',(81.4102378062637,-45.2743704641551,51.0231324337634)) ;
#14988=CARTESIAN_POINT('Ctrl Pts',(81.4471924524962,-45.5327272469311,50.9155767462735)) ;
#14989=CARTESIAN_POINT('Ctrl Pts',(81.4734523160919,-45.6499697400254,50.8349545004664)) ;
#14990=CARTESIAN_POINT('Ctrl Pts',(81.5233845132883,-45.835020200063,50.6499040404288)) ;
#14991=CARTESIAN_POINT('Ctrl Pts',(81.5504706257909,-45.9155922350857,50.5326870742094)) ;
#14992=CARTESIAN_POINT('Ctrl Pts',(81.5893583276612,-46.0231099988203,50.274427321802)) ;
#14993=CARTESIAN_POINT('Ctrl Pts',(81.6004717401017,-46.05,50.1332581893505)) ;
#14994=CARTESIAN_POINT('Ctrl Pts',(81.6004717401017,-46.05,49.8667418106495)) ;
#14995=CARTESIAN_POINT('Ctrl Pts',(81.5893583276612,-46.0231099988203,49.725572678198)) ;
#14996=CARTESIAN_POINT('Ctrl Pts',(81.5504706257909,-45.9155922350857,49.4673129257906)) ;
#14997=CARTESIAN_POINT('Ctrl Pts',(81.5233845132883,-45.835020200063,49.3500959595712)) ;
#14998=CARTESIAN_POINT('Ctrl Pts',(81.4734523160919,-45.6499697400254,49.1650454995336)) ;
#14999=CARTESIAN_POINT('Ctrl Pts',(81.4471924524962,-45.5327272469311,49.0844232537265)) ;
#15000=CARTESIAN_POINT('Ctrl Pts',(81.4102378062637,-45.2743704641551,48.9768675662366)) ;
#15001=CARTESIAN_POINT('Ctrl Pts',(81.4,-45.1331635999932,48.95)) ;
#15002=CARTESIAN_POINT('Ctrl Pts',(81.4,-45.,48.95)) ;
#15003=CARTESIAN_POINT('Origin',(87.1,45.,50.)) ;
#15004=CARTESIAN_POINT('',(87.1,45.,51.05)) ;
#15005=CARTESIAN_POINT('',(87.1,45.,48.95)) ;
#15006=CARTESIAN_POINT('Ctrl Pts',(87.1,45.,51.05)) ;
#15007=CARTESIAN_POINT('Ctrl Pts',(87.1,45.1331635999932,51.05)) ;
#15008=CARTESIAN_POINT('Ctrl Pts',(87.0897621937364,45.2743704641552,51.0231324337635)) ;
#15009=CARTESIAN_POINT('Ctrl Pts',(87.0528075475038,45.5327272469311,50.9155767462735)) ;
#15010=CARTESIAN_POINT('Ctrl Pts',(87.0265476839081,45.6499697400254,50.8349545004664)) ;
#15011=CARTESIAN_POINT('Ctrl Pts',(86.9766154867118,45.835020200063,50.6499040404288)) ;
#15012=CARTESIAN_POINT('Ctrl Pts',(86.9495293742091,45.9155922350857,50.5326870742094)) ;
#15013=CARTESIAN_POINT('Ctrl Pts',(86.9106416723389,46.0231099988203,50.274427321802)) ;
#15014=CARTESIAN_POINT('Ctrl Pts',(86.8995282598984,46.05,50.1332581893505)) ;
#15015=CARTESIAN_POINT('Ctrl Pts',(86.8995282598984,46.05,49.8667418106495)) ;
#15016=CARTESIAN_POINT('Ctrl Pts',(86.9106416723389,46.0231099988203,49.725572678198)) ;
#15017=CARTESIAN_POINT('Ctrl Pts',(86.9495293742091,45.9155922350857,49.4673129257906)) ;
#15018=CARTESIAN_POINT('Ctrl Pts',(86.9766154867118,45.835020200063,49.3500959595712)) ;
#15019=CARTESIAN_POINT('Ctrl Pts',(87.0265476839081,45.6499697400254,49.1650454995336)) ;
#15020=CARTESIAN_POINT('Ctrl Pts',(87.0528075475038,45.5327272469311,49.0844232537265)) ;
#15021=CARTESIAN_POINT('Ctrl Pts',(87.0897621937364,45.2743704641552,48.9768675662365)) ;
#15022=CARTESIAN_POINT('Ctrl Pts',(87.1,45.1331635999932,48.95)) ;
#15023=CARTESIAN_POINT('Ctrl Pts',(87.1,45.,48.95)) ;
#15024=CARTESIAN_POINT('',(81.4,45.,51.05)) ;
#15025=CARTESIAN_POINT('',(87.1,45.,51.05)) ;
#15026=CARTESIAN_POINT('',(81.4,45.,48.95)) ;
#15027=CARTESIAN_POINT('Ctrl Pts',(81.4,45.,48.95)) ;
#15028=CARTESIAN_POINT('Ctrl Pts',(81.4,45.1331635999932,48.95)) ;
#15029=CARTESIAN_POINT('Ctrl Pts',(81.4102378062637,45.2743704641552,48.9768675662365)) ;
#15030=CARTESIAN_POINT('Ctrl Pts',(81.4471924524962,45.5327272469311,49.0844232537265)) ;
#15031=CARTESIAN_POINT('Ctrl Pts',(81.4734523160919,45.6499697400254,49.1650454995336)) ;
#15032=CARTESIAN_POINT('Ctrl Pts',(81.5233845132882,45.835020200063,49.3500959595712)) ;
#15033=CARTESIAN_POINT('Ctrl Pts',(81.5504706257909,45.9155922350857,49.4673129257906)) ;
#15034=CARTESIAN_POINT('Ctrl Pts',(81.5893583276612,46.0231099988203,49.725572678198)) ;
#15035=CARTESIAN_POINT('Ctrl Pts',(81.6004717401017,46.05,49.8667418106495)) ;
#15036=CARTESIAN_POINT('Ctrl Pts',(81.6004717401017,46.05,50.1332581893505)) ;
#15037=CARTESIAN_POINT('Ctrl Pts',(81.5893583276612,46.0231099988203,50.274427321802)) ;
#15038=CARTESIAN_POINT('Ctrl Pts',(81.5504706257909,45.9155922350857,50.5326870742094)) ;
#15039=CARTESIAN_POINT('Ctrl Pts',(81.5233845132882,45.835020200063,50.6499040404288)) ;
#15040=CARTESIAN_POINT('Ctrl Pts',(81.4734523160919,45.6499697400254,50.8349545004664)) ;
#15041=CARTESIAN_POINT('Ctrl Pts',(81.4471924524962,45.5327272469311,50.9155767462735)) ;
#15042=CARTESIAN_POINT('Ctrl Pts',(81.4102378062637,45.2743704641552,51.0231324337635)) ;
#15043=CARTESIAN_POINT('Ctrl Pts',(81.4,45.1331635999932,51.05)) ;
#15044=CARTESIAN_POINT('Ctrl Pts',(81.4,45.,51.05)) ;
#15045=CARTESIAN_POINT('Ctrl Pts',(81.4,45.,51.05)) ;
#15046=CARTESIAN_POINT('Ctrl Pts',(81.4,44.8668364000068,51.05)) ;
#15047=CARTESIAN_POINT('Ctrl Pts',(81.4102378062637,44.7256295358448,51.0231324337635)) ;
#15048=CARTESIAN_POINT('Ctrl Pts',(81.4471924524962,44.4672727530689,50.9155767462735)) ;
#15049=CARTESIAN_POINT('Ctrl Pts',(81.4734523160919,44.3500302599746,50.8349545004664)) ;
#15050=CARTESIAN_POINT('Ctrl Pts',(81.5233845132882,44.164979799937,50.6499040404288)) ;
#15051=CARTESIAN_POINT('Ctrl Pts',(81.5504706257909,44.0844077649143,50.5326870742094)) ;
#15052=CARTESIAN_POINT('Ctrl Pts',(81.5893583276612,43.9768900011797,50.274427321802)) ;
#15053=CARTESIAN_POINT('Ctrl Pts',(81.6004717401017,43.95,50.1332581893505)) ;
#15054=CARTESIAN_POINT('Ctrl Pts',(81.6004717401017,43.95,50.)) ;
#15055=CARTESIAN_POINT('Ctrl Pts',(81.6004717401017,43.95,49.8667418106495)) ;
#15056=CARTESIAN_POINT('Ctrl Pts',(81.5893583276612,43.9768900011797,49.725572678198)) ;
#15057=CARTESIAN_POINT('Ctrl Pts',(81.5504706257909,44.0844077649143,49.4673129257906)) ;
#15058=CARTESIAN_POINT('Ctrl Pts',(81.5233845132882,44.164979799937,49.3500959595712)) ;
#15059=CARTESIAN_POINT('Ctrl Pts',(81.4734523160919,44.3500302599746,49.1650454995336)) ;
#15060=CARTESIAN_POINT('Ctrl Pts',(81.4471924524962,44.4672727530689,49.0844232537265)) ;
#15061=CARTESIAN_POINT('Ctrl Pts',(81.4102378062637,44.7256295358448,48.9768675662365)) ;
#15062=CARTESIAN_POINT('Ctrl Pts',(81.4,44.8668364000068,48.95)) ;
#15063=CARTESIAN_POINT('Ctrl Pts',(81.4,45.,48.95)) ;
#15064=CARTESIAN_POINT('Ctrl Pts',(87.1,45.,48.95)) ;
#15065=CARTESIAN_POINT('Ctrl Pts',(87.1,44.8668364000068,48.95)) ;
#15066=CARTESIAN_POINT('Ctrl Pts',(87.0897621937364,44.7256295358448,48.9768675662365)) ;
#15067=CARTESIAN_POINT('Ctrl Pts',(87.0528075475038,44.4672727530689,49.0844232537265)) ;
#15068=CARTESIAN_POINT('Ctrl Pts',(87.0265476839081,44.3500302599746,49.1650454995336)) ;
#15069=CARTESIAN_POINT('Ctrl Pts',(86.9766154867118,44.164979799937,49.3500959595712)) ;
#15070=CARTESIAN_POINT('Ctrl Pts',(86.9495293742091,44.0844077649143,49.4673129257906)) ;
#15071=CARTESIAN_POINT('Ctrl Pts',(86.9106416723389,43.9768900011797,49.725572678198)) ;
#15072=CARTESIAN_POINT('Ctrl Pts',(86.8995282598984,43.95,49.8667418106495)) ;
#15073=CARTESIAN_POINT('Ctrl Pts',(86.8995282598984,43.95,50.)) ;
#15074=CARTESIAN_POINT('Ctrl Pts',(86.8995282598984,43.95,50.1332581893505)) ;
#15075=CARTESIAN_POINT('Ctrl Pts',(86.9106416723389,43.9768900011797,50.274427321802)) ;
#15076=CARTESIAN_POINT('Ctrl Pts',(86.9495293742091,44.0844077649143,50.5326870742094)) ;
#15077=CARTESIAN_POINT('Ctrl Pts',(86.9766154867118,44.164979799937,50.6499040404288)) ;
#15078=CARTESIAN_POINT('Ctrl Pts',(87.0265476839081,44.3500302599746,50.8349545004664)) ;
#15079=CARTESIAN_POINT('Ctrl Pts',(87.0528075475038,44.4672727530689,50.9155767462735)) ;
#15080=CARTESIAN_POINT('Ctrl Pts',(87.0897621937364,44.7256295358448,51.0231324337635)) ;
#15081=CARTESIAN_POINT('Ctrl Pts',(87.1,44.8668364000068,51.05)) ;
#15082=CARTESIAN_POINT('Ctrl Pts',(87.1,45.,51.05)) ;
#15083=CARTESIAN_POINT('Origin',(90.25,42.5,160.)) ;
#15084=CARTESIAN_POINT('',(88.2,43.,160.)) ;
#15085=CARTESIAN_POINT('Origin',(90.25,43.,160.)) ;
#15086=CARTESIAN_POINT('',(88.2,47.,160.)) ;
#15087=CARTESIAN_POINT('',(88.2,42.5,160.)) ;
#15088=CARTESIAN_POINT('Origin',(90.25,47.,160.)) ;
#15089=CARTESIAN_POINT('Origin',(89.5,45.,163.)) ;
#15090=CARTESIAN_POINT('',(86.5,43.2507144315464,163.)) ;
#15091=CARTESIAN_POINT('',(86.5,46.7492855684536,163.)) ;
#15092=CARTESIAN_POINT('Origin',(84.25,45.,163.)) ;
#15093=CARTESIAN_POINT('',(86.5,43.,163.)) ;
#15094=CARTESIAN_POINT('',(86.5,47.,163.)) ;
#15095=CARTESIAN_POINT('',(92.5,43.,163.)) ;
#15096=CARTESIAN_POINT('',(86.5,43.,163.)) ;
#15097=CARTESIAN_POINT('',(92.5,47.,163.)) ;
#15098=CARTESIAN_POINT('',(92.5,43.,163.)) ;
#15099=CARTESIAN_POINT('',(86.5,47.,163.)) ;
#15100=CARTESIAN_POINT('',(92.5,47.,163.)) ;
#15101=CARTESIAN_POINT('',(86.5,47.,163.)) ;
#15102=CARTESIAN_POINT('Origin',(86.5,47.,157.)) ;
#15103=CARTESIAN_POINT('',(86.5,43.2507144315464,157.)) ;
#15104=CARTESIAN_POINT('',(86.5,43.2507144315464,41.)) ;
#15105=CARTESIAN_POINT('',(86.5,43.,157.)) ;
#15106=CARTESIAN_POINT('',(86.5,47.,157.)) ;
#15107=CARTESIAN_POINT('',(86.5,43.,157.)) ;
#15108=CARTESIAN_POINT('Origin',(92.5,47.,157.)) ;
#15109=CARTESIAN_POINT('',(92.5,47.,157.)) ;
#15110=CARTESIAN_POINT('',(86.5,47.,157.)) ;
#15111=CARTESIAN_POINT('',(92.5,47.,157.)) ;
#15112=CARTESIAN_POINT('',(86.5,47.,157.)) ;
#15113=CARTESIAN_POINT('',(92.5,47.,157.)) ;
#15114=CARTESIAN_POINT('Origin',(92.5,43.,157.)) ;
#15115=CARTESIAN_POINT('',(92.5,43.,157.)) ;
#15116=CARTESIAN_POINT('',(92.5,43.,157.)) ;
#15117=CARTESIAN_POINT('',(92.5,43.,157.)) ;
#15118=CARTESIAN_POINT('Origin',(86.5,43.,157.)) ;
#15119=CARTESIAN_POINT('',(86.5,43.,157.)) ;
#15120=CARTESIAN_POINT('Origin',(86.5,47.,157.)) ;
#15121=CARTESIAN_POINT('',(86.5,46.7492855684536,157.)) ;
#15122=CARTESIAN_POINT('',(86.5,46.7492855684536,41.)) ;
#15123=CARTESIAN_POINT('',(86.5,47.,157.)) ;
#15124=CARTESIAN_POINT('Origin',(89.5,45.,157.)) ;
#15125=CARTESIAN_POINT('Origin',(84.25,45.,157.)) ;
#15126=CARTESIAN_POINT('Origin',(84.25,-45.,170.)) ;
#15127=CARTESIAN_POINT('',(81.4,-45.,41.)) ;
#15128=CARTESIAN_POINT('Origin',(84.25,-45.,41.)) ;
#15129=CARTESIAN_POINT('',(81.4,-45.,170.)) ;
#15130=CARTESIAN_POINT('',(81.4,-45.,170.)) ;
#15131=CARTESIAN_POINT('',(81.4,-45.,170.)) ;
#15132=CARTESIAN_POINT('',(84.25,-42.15,170.)) ;
#15133=CARTESIAN_POINT('Origin',(84.25,-45.,170.)) ;
#15134=CARTESIAN_POINT('Origin',(84.25,-45.,170.)) ;
#15135=CARTESIAN_POINT('Origin',(84.25,-35.,170.)) ;
#15136=CARTESIAN_POINT('',(84.25,-35.,177.15)) ;
#15137=CARTESIAN_POINT('Origin',(84.25,-35.,170.)) ;
#15138=CARTESIAN_POINT('',(81.4,-35.,180.)) ;
#15139=CARTESIAN_POINT('Origin',(84.25,-35.,180.)) ;
#15140=CARTESIAN_POINT('Origin',(84.25,-35.,180.)) ;
#15141=CARTESIAN_POINT('Origin',(84.25,35.,180.)) ;
#15142=CARTESIAN_POINT('',(81.4,35.,180.)) ;
#15143=CARTESIAN_POINT('',(81.4,35.,180.)) ;
#15144=CARTESIAN_POINT('',(84.25,35.,177.15)) ;
#15145=CARTESIAN_POINT('Origin',(84.25,35.,180.)) ;
#15146=CARTESIAN_POINT('Origin',(84.25,35.,180.)) ;
#15147=CARTESIAN_POINT('Origin',(84.25,35.,170.)) ;
#15148=CARTESIAN_POINT('',(84.25,42.15,170.)) ;
#15149=CARTESIAN_POINT('Origin',(84.25,35.,170.)) ;
#15150=CARTESIAN_POINT('',(81.4,45.,170.)) ;
#15151=CARTESIAN_POINT('Origin',(84.25,45.,170.)) ;
#15152=CARTESIAN_POINT('Origin',(84.25,45.,170.)) ;
#15153=CARTESIAN_POINT('Origin',(84.25,45.,41.)) ;
#15154=CARTESIAN_POINT('',(81.4,45.,41.)) ;
#15155=CARTESIAN_POINT('',(81.4,45.,41.)) ;
#15156=CARTESIAN_POINT('',(81.4,45.,41.)) ;
#15157=CARTESIAN_POINT('Origin',(84.25,45.,41.)) ;
#15158=CARTESIAN_POINT('Origin',(84.25,-45.,41.)) ;
#15159=CARTESIAN_POINT('Origin',(84.25,45.,41.)) ;
#18729=UNCERTAINTY_MEASURE_WITH_UNIT(LENGTH_MEASURE(0.01),#18758,
'DISTANCE_ACCURACY_VALUE',
'Maximum model space distance between geometric entities at asserted c
onnectivities') ;
#18738=UNCERTAINTY_MEASURE_WITH_UNIT(LENGTH_MEASURE(0.01),#18758,
'DISTANCE_ACCURACY_VALUE',
'Maximum model space distance between geometric entities at asserted c
onnectivities') ;
#18748=(
GEOMETRIC_REPRESENTATION_CONTEXT(3)
GLOBAL_UNCERTAINTY_ASSIGNED_CONTEXT((#18729))
GLOBAL_UNIT_ASSIGNED_CONTEXT((#18758,#18760,#18761))
REPRESENTATION_CONTEXT('','3D')
) ;
#18757=(
GEOMETRIC_REPRESENTATION_CONTEXT(3)
GLOBAL_UNCERTAINTY_ASSIGNED_CONTEXT((#18738))
GLOBAL_UNIT_ASSIGNED_CONTEXT((#18758,#18760,#18761))
REPRESENTATION_CONTEXT('','3D')
) ;
#18758=(
LENGTH_UNIT()
NAMED_UNIT(*)
SI_UNIT(.MILLI.,.METRE.)
) ;
#18760=(
NAMED_UNIT(*)
PLANE_ANGLE_UNIT()
SI_UNIT($,.RADIAN.)
) ;
#18761=(
NAMED_UNIT(*)
SI_UNIT($,.STERADIAN.)
SOLID_ANGLE_UNIT()
) ;
#18771=SHAPE_DEFINITION_REPRESENTATION(#18789,#18865) ;
#18789=PRODUCT_DEFINITION_SHAPE('',$,#18884) ;
#18865=SHAPE_REPRESENTATION('',(#10171),#18748) ;
#18874=PRODUCT_DEFINITION_CONTEXT('part definition',#18930,'design') ;
#18884=PRODUCT_DEFINITION('Push Handle (chrome tube)',
'Push Handle (chrome tube)',#18902,#18874) ;
#18902=PRODUCT_DEFINITION_FORMATION('',$,#18941) ;
#18930=APPLICATION_CONTEXT(
'Core Data for Automotive Mechanical Design Process') ;
#18931=PRODUCT_CONTEXT('part definition',#18930,'mechanical') ;
#18941=PRODUCT('Push Handle (chrome tube)','Push Handle (chrome tube)',$,
(#18931)) ;
#18959=PRESENTATION_STYLE_ASSIGNMENT((#18977)) ;
#18977=SURFACE_STYLE_USAGE(.BOTH.,#18995) ;
#18995=SURFACE_SIDE_STYLE('',(#19013)) ;
#19013=SURFACE_STYLE_FILL_AREA(#19031) ;
#19031=FILL_AREA_STYLE(
'MAS-253 Metallic Sheet - Push Handle (chrome tube)',(#19049)) ;
#19049=FILL_AREA_STYLE_COLOUR(
'MAS-253 Metallic Sheet - Push Handle (chrome tube)',#19067) ;
#19067=COLOUR_RGB('MAS-253 Metallic Sheet - Push Handle (chrome tube)', 0.40784314, 0.44705882, 0.49803922) ;
ENDSEC;
END-ISO-10303-21;
